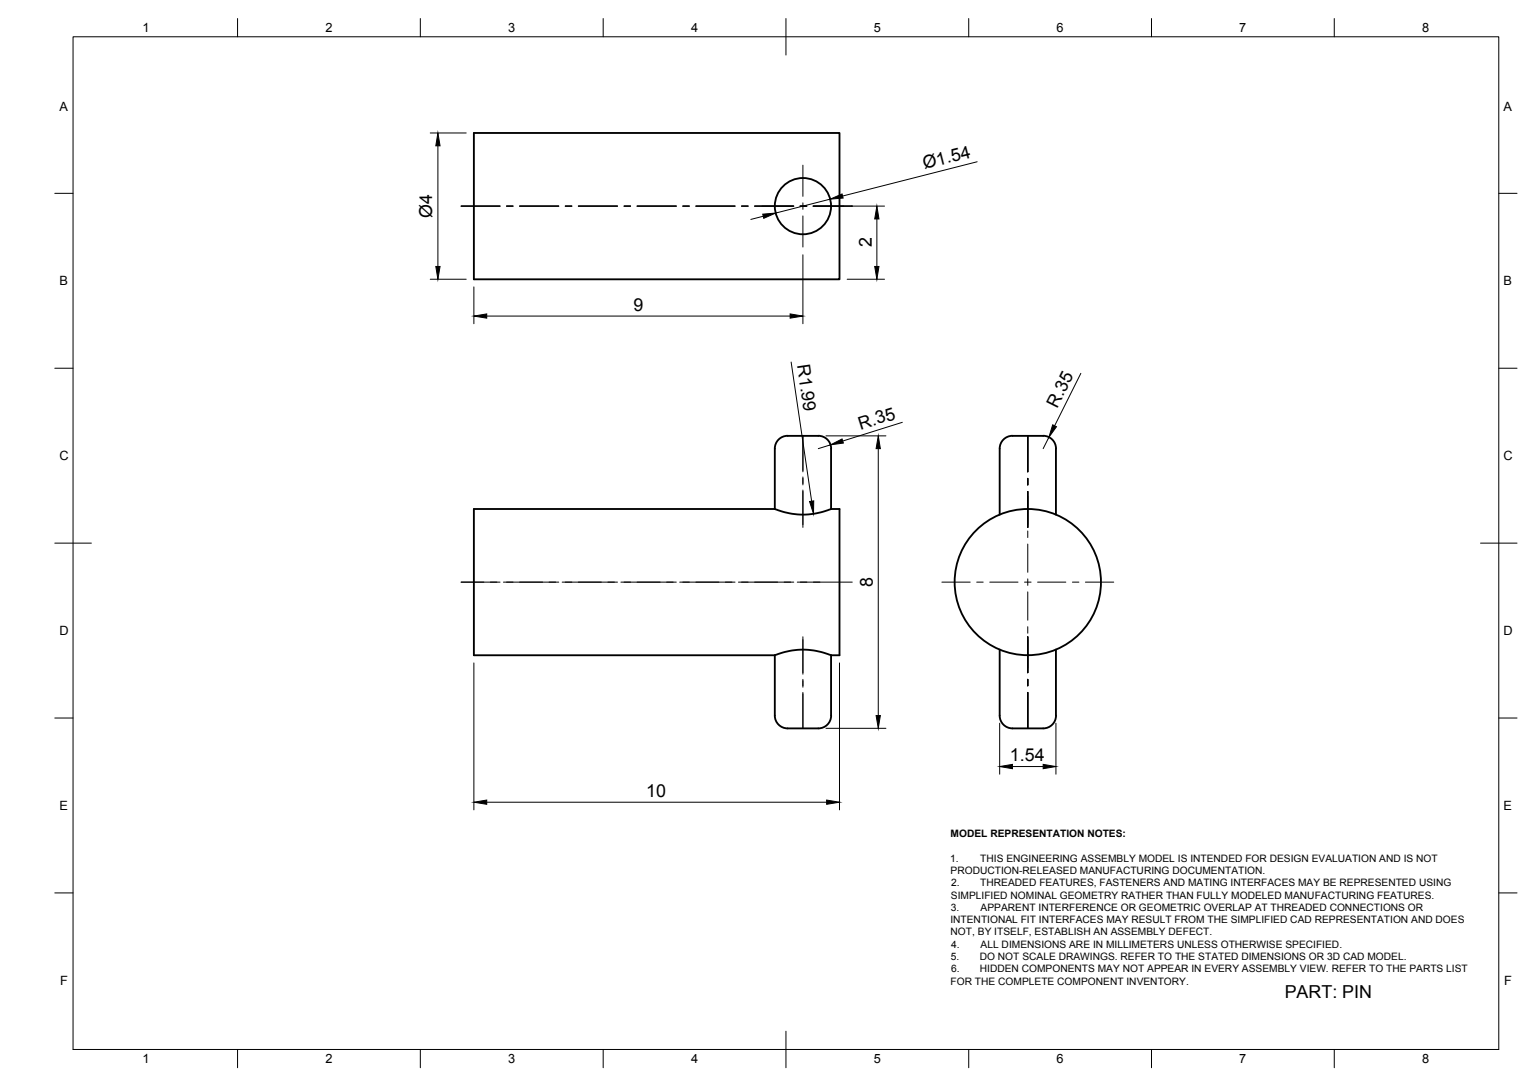
ISO-10303-21;
HEADER;
/* Generated by software containing ST-Developer
 * from STEP Tools, Inc. (www.steptools.com) 
 */

FILE_DESCRIPTION(
/* description */ (''),
/* implementation_level */ '2;1');

FILE_NAME(
/* name */ 'Pin.step',
/* time_stamp */ '2026-10-04T15:18:51-07:00',
/* author */ (''),
/* organization */ (''),
/* preprocessor_version */ 'ST-DEVELOPER v20.2',
/* originating_system */ 'Autodesk Translation Framework v15.15.0.0',
/* authorisation */ '');

FILE_SCHEMA (('AUTOMOTIVE_DESIGN { 1 0 10303 214 3 1 1 }'));
ENDSEC;

DATA;
#10=MECHANICAL_DESIGN_GEOMETRIC_PRESENTATION_REPRESENTATION('',(#75),#9891);
#47=B_SPLINE_CURVE_WITH_KNOTS('',3,(#8554,#8555,#8556,#8557,#8558,#8559,
#8560,#8561,#8562,#8563,#8564,#8565,#8566,#8567,#8568,#8569,#8570,#8571,
#8572,#8573,#8574,#8575,#8576,#8577,#8578,#8579),.UNSPECIFIED.,.F.,.F.,
(4,2,2,2,2,2,2,2,2,2,2,2,4),(0.,0.0293489859798306,0.0586979719596612,0.0880217900278663,
0.117345608096071,0.146669426164276,0.175993244232481,0.205342230212312,
0.234691216192143,0.264040202171973,0.293389188151804,0.322713006220009,
0.352036824288214),.UNSPECIFIED.);
#48=B_SPLINE_CURVE_WITH_KNOTS('',3,(#8580,#8581,#8582,#8583,#8584,#8585,
#8586,#8587,#8588,#8589),.UNSPECIFIED.,.F.,.F.,(4,2,2,2,4),(0.352036824288214,
0.381360642356419,0.410684460424624,0.440033446404455,0.469382432384286),
 .UNSPECIFIED.);
#49=B_SPLINE_CURVE_WITH_KNOTS('',3,(#8602,#8603,#8604,#8605,#8606,#8607,
#8608,#8609,#8610,#8611),.UNSPECIFIED.,.F.,.F.,(4,2,2,2,4),(0.,0.0293489859798306,
0.0586979719596612,0.0880217900278663,0.117345608096071),.UNSPECIFIED.);
#50=B_SPLINE_CURVE_WITH_KNOTS('',3,(#8613,#8614,#8615,#8616,#8617,#8618,
#8619,#8620,#8621,#8622),.UNSPECIFIED.,.F.,.F.,(4,2,2,2,4),(0.352036824288214,
0.381360642356419,0.410684460424624,0.440033446404455,0.469382432384285),
 .UNSPECIFIED.);
#51=B_SPLINE_CURVE_WITH_KNOTS('',3,(#8623,#8624,#8625,#8626,#8627,#8628,
#8629,#8630,#8631,#8632,#8633,#8634,#8635,#8636,#8637,#8638,#8639,#8640),
 .UNSPECIFIED.,.F.,.F.,(4,2,2,2,2,2,2,2,4),(0.117345608096071,0.146669426164276,
0.175993244232481,0.205342230212312,0.234691216192143,0.264040202171973,
0.293389188151804,0.322713006220009,0.352036824288214),.UNSPECIFIED.);
#56=SHAPE_REPRESENTATION_RELATIONSHIP('SRR','None',#9927,#64);
#64=ADVANCED_BREP_SHAPE_REPRESENTATION('',(#89),#9887);
#75=STYLED_ITEM('',(#9972),#89);
#89=MANIFOLD_SOLID_BREP('Body1',#5623);
#125=FACE_BOUND('',#867,.T.);
#198=PLANE('',#5935);
#199=PLANE('',#5942);
#200=PLANE('',#5943);
#201=PLANE('',#5947);
#358=TOROIDAL_SURFACE('',#5929,0.420000000000005,0.35);
#359=TOROIDAL_SURFACE('',#5936,0.420000000000005,0.35);
#500=FACE_OUTER_BOUND('',#859,.T.);
#501=FACE_OUTER_BOUND('',#860,.T.);
#502=FACE_OUTER_BOUND('',#861,.T.);
#503=FACE_OUTER_BOUND('',#862,.T.);
#504=FACE_OUTER_BOUND('',#863,.T.);
#505=FACE_OUTER_BOUND('',#864,.T.);
#506=FACE_OUTER_BOUND('',#865,.T.);
#507=FACE_OUTER_BOUND('',#866,.T.);
#508=FACE_OUTER_BOUND('',#868,.T.);
#859=EDGE_LOOP('',(#3978,#3979,#3980,#3981,#3982));
#860=EDGE_LOOP('',(#3983,#3984,#3985,#3986,#3987,#3988));
#861=EDGE_LOOP('',(#3989));
#862=EDGE_LOOP('',(#3990,#3991,#3992,#3993,#3994));
#863=EDGE_LOOP('',(#3995,#3996,#3997,#3998,#3999,#4000,#4001));
#864=EDGE_LOOP('',(#4002));
#865=EDGE_LOOP('',(#4003));
#866=EDGE_LOOP('',(#4004,#4005,#4006,#4007,#4008,#4009,#4010,#4011,#4012));
#867=EDGE_LOOP('',(#4013,#4014));
#868=EDGE_LOOP('',(#4015));
#1183=LINE('',#8552,#1647);
#1184=LINE('',#8641,#1648);
#1185=LINE('',#8649,#1649);
#1186=LINE('',#8650,#1650);
#1647=VECTOR('',#6854,0.770000000000005);
#1648=VECTOR('',#6869,0.770000000000005);
#1649=VECTOR('',#6880,1.99999999999999);
#1650=VECTOR('',#6881,1.99999999999999);
#2171=CIRCLE('',#5930,0.420000000000005);
#2172=CIRCLE('',#5931,0.35);
#2173=CIRCLE('',#5932,0.770000000000005);
#2174=CIRCLE('',#5933,0.770000000000005);
#2175=CIRCLE('',#5937,0.420000000000005);
#2176=CIRCLE('',#5938,0.35);
#2177=CIRCLE('',#5939,0.770000000000005);
#2178=CIRCLE('',#5940,0.770000000000005);
#2179=CIRCLE('',#5944,1.99999999999999);
#2180=CIRCLE('',#5946,1.99999999999999);
#2467=VERTEX_POINT('',#8543);
#2468=VERTEX_POINT('',#8545);
#2469=VERTEX_POINT('',#8547);
#2470=VERTEX_POINT('',#8551);
#2471=VERTEX_POINT('',#8553);
#2472=VERTEX_POINT('',#8592);
#2473=VERTEX_POINT('',#8594);
#2474=VERTEX_POINT('',#8596);
#2475=VERTEX_POINT('',#8600);
#2476=VERTEX_POINT('',#8601);
#2477=VERTEX_POINT('',#8612);
#2478=VERTEX_POINT('',#8644);
#2479=VERTEX_POINT('',#8647);
#3034=EDGE_CURVE('',#2467,#2467,#2171,.T.);
#3035=EDGE_CURVE('',#2467,#2468,#2172,.T.);
#3036=EDGE_CURVE('',#2468,#2469,#2173,.T.);
#3037=EDGE_CURVE('',#2469,#2468,#2174,.T.);
#3038=EDGE_CURVE('',#2469,#2470,#1183,.T.);
#3039=EDGE_CURVE('',#2471,#2470,#47,.T.);
#3040=EDGE_CURVE('',#2470,#2471,#48,.T.);
#3041=EDGE_CURVE('',#2472,#2472,#2175,.T.);
#3042=EDGE_CURVE('',#2472,#2473,#2176,.T.);
#3043=EDGE_CURVE('',#2473,#2474,#2177,.T.);
#3044=EDGE_CURVE('',#2474,#2473,#2178,.T.);
#3045=EDGE_CURVE('',#2475,#2476,#49,.T.);
#3046=EDGE_CURVE('',#2477,#2475,#50,.T.);
#3047=EDGE_CURVE('',#2476,#2477,#51,.T.);
#3048=EDGE_CURVE('',#2476,#2474,#1184,.T.);
#3049=EDGE_CURVE('',#2478,#2478,#2179,.T.);
#3050=EDGE_CURVE('',#2479,#2479,#2180,.T.);
#3051=EDGE_CURVE('',#2479,#2476,#1185,.T.);
#3052=EDGE_CURVE('',#2477,#2478,#1186,.T.);
#3978=ORIENTED_EDGE('',*,*,#3034,.T.);
#3979=ORIENTED_EDGE('',*,*,#3035,.T.);
#3980=ORIENTED_EDGE('',*,*,#3036,.T.);
#3981=ORIENTED_EDGE('',*,*,#3037,.T.);
#3982=ORIENTED_EDGE('',*,*,#3035,.F.);
#3983=ORIENTED_EDGE('',*,*,#3037,.F.);
#3984=ORIENTED_EDGE('',*,*,#3038,.T.);
#3985=ORIENTED_EDGE('',*,*,#3039,.F.);
#3986=ORIENTED_EDGE('',*,*,#3040,.F.);
#3987=ORIENTED_EDGE('',*,*,#3038,.F.);
#3988=ORIENTED_EDGE('',*,*,#3036,.F.);
#3989=ORIENTED_EDGE('',*,*,#3034,.F.);
#3990=ORIENTED_EDGE('',*,*,#3041,.T.);
#3991=ORIENTED_EDGE('',*,*,#3042,.T.);
#3992=ORIENTED_EDGE('',*,*,#3043,.T.);
#3993=ORIENTED_EDGE('',*,*,#3044,.T.);
#3994=ORIENTED_EDGE('',*,*,#3042,.F.);
#3995=ORIENTED_EDGE('',*,*,#3045,.F.);
#3996=ORIENTED_EDGE('',*,*,#3046,.F.);
#3997=ORIENTED_EDGE('',*,*,#3047,.F.);
#3998=ORIENTED_EDGE('',*,*,#3048,.T.);
#3999=ORIENTED_EDGE('',*,*,#3043,.F.);
#4000=ORIENTED_EDGE('',*,*,#3044,.F.);
#4001=ORIENTED_EDGE('',*,*,#3048,.F.);
#4002=ORIENTED_EDGE('',*,*,#3041,.F.);
#4003=ORIENTED_EDGE('',*,*,#3049,.T.);
#4004=ORIENTED_EDGE('',*,*,#3050,.F.);
#4005=ORIENTED_EDGE('',*,*,#3051,.T.);
#4006=ORIENTED_EDGE('',*,*,#3047,.T.);
#4007=ORIENTED_EDGE('',*,*,#3052,.T.);
#4008=ORIENTED_EDGE('',*,*,#3049,.F.);
#4009=ORIENTED_EDGE('',*,*,#3052,.F.);
#4010=ORIENTED_EDGE('',*,*,#3046,.T.);
#4011=ORIENTED_EDGE('',*,*,#3045,.T.);
#4012=ORIENTED_EDGE('',*,*,#3051,.F.);
#4013=ORIENTED_EDGE('',*,*,#3039,.T.);
#4014=ORIENTED_EDGE('',*,*,#3040,.T.);
#4015=ORIENTED_EDGE('',*,*,#3050,.T.);
#5222=CYLINDRICAL_SURFACE('',#5934,0.770000000000005);
#5223=CYLINDRICAL_SURFACE('',#5941,0.770000000000005);
#5224=CYLINDRICAL_SURFACE('',#5945,1.99999999999999);
#5379=ADVANCED_FACE('',(#500),#358,.T.);
#5380=ADVANCED_FACE('',(#501),#5222,.T.);
#5381=ADVANCED_FACE('',(#502),#198,.T.);
#5382=ADVANCED_FACE('',(#503),#359,.T.);
#5383=ADVANCED_FACE('',(#504),#5223,.T.);
#5384=ADVANCED_FACE('',(#505),#199,.F.);
#5385=ADVANCED_FACE('',(#506),#200,.F.);
#5386=ADVANCED_FACE('',(#507,#125),#5224,.T.);
#5387=ADVANCED_FACE('',(#508),#201,.T.);
#5623=CLOSED_SHELL('',(#5379,#5380,#5381,#5382,#5383,#5384,#5385,#5386,
#5387));
#5928=AXIS2_PLACEMENT_3D('',#8541,#6840,#6841);
#5929=AXIS2_PLACEMENT_3D('',#8542,#6842,#6843);
#5930=AXIS2_PLACEMENT_3D('',#8544,#6844,#6845);
#5931=AXIS2_PLACEMENT_3D('',#8546,#6846,#6847);
#5932=AXIS2_PLACEMENT_3D('',#8548,#6848,#6849);
#5933=AXIS2_PLACEMENT_3D('',#8549,#6850,#6851);
#5934=AXIS2_PLACEMENT_3D('',#8550,#6852,#6853);
#5935=AXIS2_PLACEMENT_3D('',#8590,#6855,#6856);
#5936=AXIS2_PLACEMENT_3D('',#8591,#6857,#6858);
#5937=AXIS2_PLACEMENT_3D('',#8593,#6859,#6860);
#5938=AXIS2_PLACEMENT_3D('',#8595,#6861,#6862);
#5939=AXIS2_PLACEMENT_3D('',#8597,#6863,#6864);
#5940=AXIS2_PLACEMENT_3D('',#8598,#6865,#6866);
#5941=AXIS2_PLACEMENT_3D('',#8599,#6867,#6868);
#5942=AXIS2_PLACEMENT_3D('',#8642,#6870,#6871);
#5943=AXIS2_PLACEMENT_3D('',#8643,#6872,#6873);
#5944=AXIS2_PLACEMENT_3D('',#8645,#6874,#6875);
#5945=AXIS2_PLACEMENT_3D('',#8646,#6876,#6877);
#5946=AXIS2_PLACEMENT_3D('',#8648,#6878,#6879);
#5947=AXIS2_PLACEMENT_3D('',#8651,#6882,#6883);
#6840=DIRECTION('axis',(0.,0.,1.));
#6841=DIRECTION('refdir',(1.,0.,0.));
#6842=DIRECTION('center_axis',(1.,0.,0.));
#6843=DIRECTION('ref_axis',(0.,0.,-1.));
#6844=DIRECTION('center_axis',(-1.,0.,0.));
#6845=DIRECTION('ref_axis',(0.,1.,0.));
#6846=DIRECTION('center_axis',(0.,-1.,0.));
#6847=DIRECTION('ref_axis',(0.,0.,1.));
#6848=DIRECTION('center_axis',(1.,0.,0.));
#6849=DIRECTION('ref_axis',(0.,1.,0.));
#6850=DIRECTION('center_axis',(1.,0.,0.));
#6851=DIRECTION('ref_axis',(0.,1.,0.));
#6852=DIRECTION('center_axis',(1.,0.,0.));
#6853=DIRECTION('ref_axis',(0.,1.,0.));
#6854=DIRECTION('',(-1.,0.,0.));
#6855=DIRECTION('center_axis',(1.,0.,0.));
#6856=DIRECTION('ref_axis',(0.,1.,0.));
#6857=DIRECTION('center_axis',(-1.,0.,0.));
#6858=DIRECTION('ref_axis',(0.,0.,1.));
#6859=DIRECTION('center_axis',(1.,0.,0.));
#6860=DIRECTION('ref_axis',(0.,1.,0.));
#6861=DIRECTION('center_axis',(0.,-1.,0.));
#6862=DIRECTION('ref_axis',(0.,0.,-1.));
#6863=DIRECTION('center_axis',(-1.,0.,0.));
#6864=DIRECTION('ref_axis',(0.,1.,0.));
#6865=DIRECTION('center_axis',(-1.,0.,0.));
#6866=DIRECTION('ref_axis',(0.,1.,0.));
#6867=DIRECTION('center_axis',(1.,0.,0.));
#6868=DIRECTION('ref_axis',(0.,1.,0.));
#6869=DIRECTION('',(-1.,0.,0.));
#6870=DIRECTION('center_axis',(1.,0.,0.));
#6871=DIRECTION('ref_axis',(0.,1.,0.));
#6872=DIRECTION('center_axis',(-8.32667268468864E-17,-1.,-2.13821176807379E-50));
#6873=DIRECTION('ref_axis',(1.,-8.32667268468864E-17,-1.5395124730131E-48));
#6874=DIRECTION('center_axis',(8.32667268468864E-17,1.,2.13821176807379E-50));
#6875=DIRECTION('ref_axis',(1.,-8.32667268468864E-17,-1.5395124730131E-48));
#6876=DIRECTION('center_axis',(-6.93889390390723E-17,-1.,0.));
#6877=DIRECTION('ref_axis',(1.,-6.93889390390723E-17,-1.5395124730131E-48));
#6878=DIRECTION('center_axis',(-8.32667268468864E-17,-1.,-2.13821176807379E-50));
#6879=DIRECTION('ref_axis',(1.,-8.32667268468864E-17,-1.5395124730131E-48));
#6880=DIRECTION('',(6.93889390390723E-17,1.,0.));
#6881=DIRECTION('',(6.93889390390723E-17,1.,0.));
#6882=DIRECTION('center_axis',(-8.32667268468864E-17,-1.,-2.13821176807379E-50));
#6883=DIRECTION('ref_axis',(1.,-8.32667268468864E-17,-1.5395124730131E-48));
#8541=CARTESIAN_POINT('',(0.,0.,0.));
#8542=CARTESIAN_POINT('Origin',(3.65,-7.00000000000001,86.8));
#8543=CARTESIAN_POINT('',(4.,-7.00000000000001,87.22));
#8544=CARTESIAN_POINT('Origin',(4.,-7.00000000000001,86.8));
#8545=CARTESIAN_POINT('',(3.65,-7.00000000000001,87.57));
#8546=CARTESIAN_POINT('Origin',(3.65,-7.00000000000001,87.22));
#8547=CARTESIAN_POINT('',(3.65,-7.77000000000001,86.8));
#8548=CARTESIAN_POINT('Origin',(3.65,-7.00000000000001,86.8));
#8549=CARTESIAN_POINT('Origin',(3.65,-7.00000000000001,86.8));
#8550=CARTESIAN_POINT('Origin',(0.,-7.00000000000001,86.8));
#8551=CARTESIAN_POINT('',(1.99999999999999,-7.77000000000002,86.8));
#8552=CARTESIAN_POINT('',(0.,-7.77000000000002,86.8));
#8553=CARTESIAN_POINT('',(1.84583314522196,-7.00000000000001,87.57));
#8554=CARTESIAN_POINT('Ctrl Pts',(1.84583314522195,-7.00000000000001,87.57));
#8555=CARTESIAN_POINT('Ctrl Pts',(1.84583314522195,-6.90217004673391,87.57));
#8556=CARTESIAN_POINT('Ctrl Pts',(1.854432195632,-6.79861108012537,87.5502407729135));
#8557=CARTESIAN_POINT('Ctrl Pts',(1.88442049625666,-6.60925764081413,87.4713711812985));
#8558=CARTESIAN_POINT('Ctrl Pts',(1.90526976397196,-6.52335991547568,87.412304358503));
#8559=CARTESIAN_POINT('Ctrl Pts',(1.94363570580007,-6.38775381022663,87.2766982532539));
#8560=CARTESIAN_POINT('Ctrl Pts',(1.96378848031407,-6.32864270522496,87.1907782243559));
#8561=CARTESIAN_POINT('Ctrl Pts',(1.99214343577073,-6.24973944011141,87.0013388884702));
#8562=CARTESIAN_POINT('Ctrl Pts',(1.99999999999999,-6.23000000000001,86.8977460602273));
#8563=CARTESIAN_POINT('Ctrl Pts',(1.99999999999999,-6.23000000000001,86.7022539397726));
#8564=CARTESIAN_POINT('Ctrl Pts',(1.99214343577073,-6.24973944011141,86.5986611115298));
#8565=CARTESIAN_POINT('Ctrl Pts',(1.96378848031407,-6.32864270522496,86.4092217756441));
#8566=CARTESIAN_POINT('Ctrl Pts',(1.94363570580007,-6.38775381022663,86.3233017467461));
#8567=CARTESIAN_POINT('Ctrl Pts',(1.90526976397196,-6.52335991547568,86.187695641497));
#8568=CARTESIAN_POINT('Ctrl Pts',(1.88442049625666,-6.60925764081413,86.1286288187015));
#8569=CARTESIAN_POINT('Ctrl Pts',(1.854432195632,-6.79861108012537,86.0497592270865));
#8570=CARTESIAN_POINT('Ctrl Pts',(1.84583314522195,-6.90217004673391,86.03));
#8571=CARTESIAN_POINT('Ctrl Pts',(1.84583314522195,-7.09782995326611,86.03));
#8572=CARTESIAN_POINT('Ctrl Pts',(1.854432195632,-7.20138891987465,86.0497592270865));
#8573=CARTESIAN_POINT('Ctrl Pts',(1.88442049625666,-7.39074235918589,86.1286288187015));
#8574=CARTESIAN_POINT('Ctrl Pts',(1.90526976397196,-7.47664008452434,86.187695641497));
#8575=CARTESIAN_POINT('Ctrl Pts',(1.94363570580007,-7.61224618977339,86.3233017467461));
#8576=CARTESIAN_POINT('Ctrl Pts',(1.96378848031406,-7.67135729477505,86.4092217756441));
#8577=CARTESIAN_POINT('Ctrl Pts',(1.99214343577073,-7.75026055988861,86.5986611115297));
#8578=CARTESIAN_POINT('Ctrl Pts',(1.99999999999999,-7.77000000000002,86.7022539397726));
#8579=CARTESIAN_POINT('Ctrl Pts',(1.99999999999999,-7.77000000000002,86.8));
#8580=CARTESIAN_POINT('Ctrl Pts',(1.99999999999999,-7.77000000000002,86.8));
#8581=CARTESIAN_POINT('Ctrl Pts',(1.99999999999999,-7.77000000000002,86.8977460602273));
#8582=CARTESIAN_POINT('Ctrl Pts',(1.99214343577073,-7.75026055988861,87.0013388884702));
#8583=CARTESIAN_POINT('Ctrl Pts',(1.96378848031407,-7.67135729477507,87.1907782243559));
#8584=CARTESIAN_POINT('Ctrl Pts',(1.94363570580007,-7.61224618977339,87.2766982532539));
#8585=CARTESIAN_POINT('Ctrl Pts',(1.90526976397196,-7.47664008452434,87.412304358503));
#8586=CARTESIAN_POINT('Ctrl Pts',(1.88442049625666,-7.39074235918589,87.4713711812985));
#8587=CARTESIAN_POINT('Ctrl Pts',(1.854432195632,-7.20138891987465,87.5502407729135));
#8588=CARTESIAN_POINT('Ctrl Pts',(1.84583314522195,-7.09782995326611,87.57));
#8589=CARTESIAN_POINT('Ctrl Pts',(1.84583314522195,-7.00000000000001,87.57));
#8590=CARTESIAN_POINT('Origin',(4.,-7.00000000000001,86.8));
#8591=CARTESIAN_POINT('Origin',(-3.65,-7.00000000000001,86.8));
#8592=CARTESIAN_POINT('',(-4.,-7.00000000000001,86.38));
#8593=CARTESIAN_POINT('Origin',(-4.,-7.00000000000001,86.8));
#8594=CARTESIAN_POINT('',(-3.65,-7.00000000000001,86.03));
#8595=CARTESIAN_POINT('Origin',(-3.65,-7.00000000000001,86.38));
#8596=CARTESIAN_POINT('',(-3.65,-7.77000000000001,86.8));
#8597=CARTESIAN_POINT('Origin',(-3.65,-7.00000000000001,86.8));
#8598=CARTESIAN_POINT('Origin',(-3.65,-7.00000000000001,86.8));
#8599=CARTESIAN_POINT('Origin',(0.,-7.00000000000001,86.8));
#8600=CARTESIAN_POINT('',(-1.84583314522196,-7.00000000000001,87.57));
#8601=CARTESIAN_POINT('',(-1.99999999999999,-7.77000000000002,86.8));
#8602=CARTESIAN_POINT('Ctrl Pts',(-1.84583314522195,-7.00000000000001,87.57));
#8603=CARTESIAN_POINT('Ctrl Pts',(-1.84583314522195,-7.09782995326611,87.57));
#8604=CARTESIAN_POINT('Ctrl Pts',(-1.854432195632,-7.20138891987465,87.5502407729135));
#8605=CARTESIAN_POINT('Ctrl Pts',(-1.88442049625666,-7.39074235918589,87.4713711812985));
#8606=CARTESIAN_POINT('Ctrl Pts',(-1.90526976397196,-7.47664008452434,87.412304358503));
#8607=CARTESIAN_POINT('Ctrl Pts',(-1.94363570580007,-7.61224618977339,87.2766982532539));
#8608=CARTESIAN_POINT('Ctrl Pts',(-1.96378848031407,-7.67135729477507,87.1907782243559));
#8609=CARTESIAN_POINT('Ctrl Pts',(-1.99214343577073,-7.75026055988861,87.0013388884702));
#8610=CARTESIAN_POINT('Ctrl Pts',(-1.99999999999999,-7.77000000000002,86.8977460602273));
#8611=CARTESIAN_POINT('Ctrl Pts',(-1.99999999999999,-7.77000000000002,86.8));
#8612=CARTESIAN_POINT('',(-1.99999999999999,-6.23,86.8));
#8613=CARTESIAN_POINT('Ctrl Pts',(-1.99999999999999,-6.23000000000001,86.8));
#8614=CARTESIAN_POINT('Ctrl Pts',(-1.99999999999999,-6.23000000000001,86.8977460602273));
#8615=CARTESIAN_POINT('Ctrl Pts',(-1.99214343577073,-6.24973944011141,87.0013388884702));
#8616=CARTESIAN_POINT('Ctrl Pts',(-1.96378848031407,-6.32864270522496,87.1907782243559));
#8617=CARTESIAN_POINT('Ctrl Pts',(-1.94363570580007,-6.38775381022663,87.2766982532539));
#8618=CARTESIAN_POINT('Ctrl Pts',(-1.90526976397196,-6.52335991547568,87.412304358503));
#8619=CARTESIAN_POINT('Ctrl Pts',(-1.88442049625666,-6.60925764081413,87.4713711812985));
#8620=CARTESIAN_POINT('Ctrl Pts',(-1.854432195632,-6.79861108012537,87.5502407729135));
#8621=CARTESIAN_POINT('Ctrl Pts',(-1.84583314522195,-6.90217004673391,87.57));
#8622=CARTESIAN_POINT('Ctrl Pts',(-1.84583314522195,-7.00000000000001,87.57));
#8623=CARTESIAN_POINT('Ctrl Pts',(-1.99999999999999,-7.77000000000002,86.8));
#8624=CARTESIAN_POINT('Ctrl Pts',(-1.99999999999999,-7.77000000000002,86.7022539397726));
#8625=CARTESIAN_POINT('Ctrl Pts',(-1.99214343577073,-7.75026055988861,86.5986611115298));
#8626=CARTESIAN_POINT('Ctrl Pts',(-1.96378848031407,-7.67135729477507,86.4092217756441));
#8627=CARTESIAN_POINT('Ctrl Pts',(-1.94363570580007,-7.61224618977339,86.3233017467461));
#8628=CARTESIAN_POINT('Ctrl Pts',(-1.90526976397196,-7.47664008452434,86.187695641497));
#8629=CARTESIAN_POINT('Ctrl Pts',(-1.88442049625666,-7.39074235918589,86.1286288187015));
#8630=CARTESIAN_POINT('Ctrl Pts',(-1.854432195632,-7.20138891987465,86.0497592270865));
#8631=CARTESIAN_POINT('Ctrl Pts',(-1.84583314522195,-7.09782995326611,86.03));
#8632=CARTESIAN_POINT('Ctrl Pts',(-1.84583314522195,-6.90217004673391,86.03));
#8633=CARTESIAN_POINT('Ctrl Pts',(-1.854432195632,-6.79861108012537,86.0497592270865));
#8634=CARTESIAN_POINT('Ctrl Pts',(-1.88442049625666,-6.60925764081413,86.1286288187015));
#8635=CARTESIAN_POINT('Ctrl Pts',(-1.90526976397196,-6.52335991547568,86.187695641497));
#8636=CARTESIAN_POINT('Ctrl Pts',(-1.94363570580007,-6.38775381022663,86.3233017467461));
#8637=CARTESIAN_POINT('Ctrl Pts',(-1.96378848031407,-6.32864270522496,86.4092217756441));
#8638=CARTESIAN_POINT('Ctrl Pts',(-1.99214343577073,-6.24973944011141,86.5986611115298));
#8639=CARTESIAN_POINT('Ctrl Pts',(-1.99999999999999,-6.23000000000001,86.7022539397726));
#8640=CARTESIAN_POINT('Ctrl Pts',(-1.99999999999999,-6.23000000000001,86.8));
#8641=CARTESIAN_POINT('',(0.,-7.77000000000002,86.8));
#8642=CARTESIAN_POINT('Origin',(-4.,-7.00000000000001,86.8));
#8643=CARTESIAN_POINT('Origin',(1.0547118830044E-15,1.99999999999999,86.8));
#8644=CARTESIAN_POINT('',(-1.99999999999999,1.99999999999999,86.8));
#8645=CARTESIAN_POINT('Origin',(9.20093280439024E-16,1.99999999999999,86.8));
#8646=CARTESIAN_POINT('Origin',(3.64981768126446E-16,-4.00000000000001,
86.8));
#8647=CARTESIAN_POINT('',(-1.99999999999999,-8.00000000000001,86.8));
#8648=CARTESIAN_POINT('Origin',(8.74260119701567E-17,-8.00000000000001,
86.8));
#8649=CARTESIAN_POINT('',(-1.99999999999999,-4.00000000000001,86.8));
#8650=CARTESIAN_POINT('',(-1.99999999999999,-4.00000000000001,86.8));
#8651=CARTESIAN_POINT('Origin',(2.22044614535531E-16,-8.00000000000001,
86.8));
#9877=UNCERTAINTY_MEASURE_WITH_UNIT(LENGTH_MEASURE(0.01),#9892,
'DISTANCE_ACCURACY_VALUE',
'Maximum model space distance between geometric entities at asserted c
onnectivities');
#9881=UNCERTAINTY_MEASURE_WITH_UNIT(LENGTH_MEASURE(0.01),#9892,
'DISTANCE_ACCURACY_VALUE',
'Maximum model space distance between geometric entities at asserted c
onnectivities');
#9887=(
GEOMETRIC_REPRESENTATION_CONTEXT(3)
GLOBAL_UNCERTAINTY_ASSIGNED_CONTEXT((#9877))
GLOBAL_UNIT_ASSIGNED_CONTEXT((#9892,#9894,#9895))
REPRESENTATION_CONTEXT('','3D')
);
#9891=(
GEOMETRIC_REPRESENTATION_CONTEXT(3)
GLOBAL_UNCERTAINTY_ASSIGNED_CONTEXT((#9881))
GLOBAL_UNIT_ASSIGNED_CONTEXT((#9892,#9894,#9895))
REPRESENTATION_CONTEXT('','3D')
);
#9892=(
LENGTH_UNIT()
NAMED_UNIT(*)
SI_UNIT(.MILLI.,.METRE.)
);
#9894=(
NAMED_UNIT(*)
PLANE_ANGLE_UNIT()
SI_UNIT($,.RADIAN.)
);
#9895=(
NAMED_UNIT(*)
SI_UNIT($,.STERADIAN.)
SOLID_ANGLE_UNIT()
);
#9901=SHAPE_DEFINITION_REPRESENTATION(#9910,#9927);
#9910=PRODUCT_DEFINITION_SHAPE('',$,#9937);
#9927=SHAPE_REPRESENTATION('',(#5928),#9887);
#9931=PRODUCT_DEFINITION_CONTEXT('part definition',#9960,'design');
#9937=PRODUCT_DEFINITION('Pin','Pin',#9946,#9931);
#9946=PRODUCT_DEFINITION_FORMATION('',$,#9967);
#9960=APPLICATION_CONTEXT(
'Core Data for Automotive Mechanical Design Process');
#9961=PRODUCT_CONTEXT('part definition',#9960,'mechanical');
#9967=PRODUCT('Pin','Pin',$,(#9961));
#9972=PRESENTATION_STYLE_ASSIGNMENT((#9977));
#9977=SURFACE_STYLE_USAGE(.BOTH.,#9982);
#9982=SURFACE_SIDE_STYLE('',(#9987));
#9987=SURFACE_STYLE_FILL_AREA(#9992);
#9992=FILL_AREA_STYLE('Opaque(160,160,160)',(#9997));
#9997=FILL_AREA_STYLE_COLOUR('Opaque(160,160,160)',#10002);
#10002=COLOUR_RGB('Opaque(160,160,160)', 0.09019608, 0.27058824, 0.51372549);
ENDSEC;
END-ISO-10303-21;
